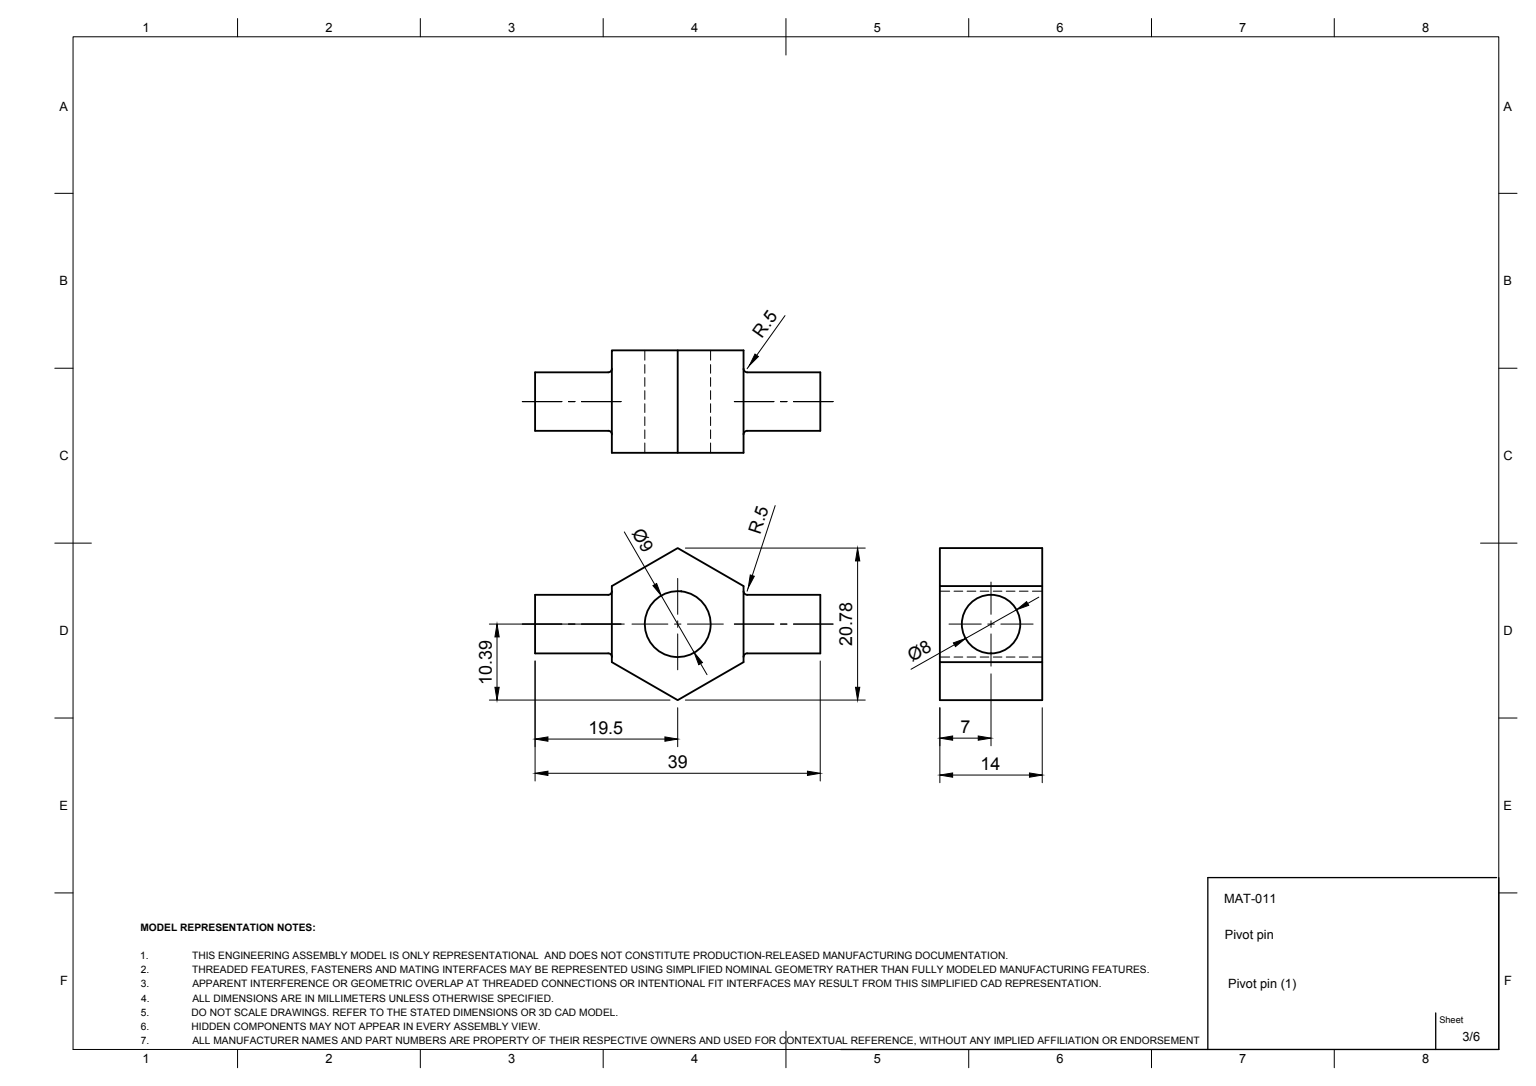
ISO-10303-21;
HEADER;
/* Generated by software containing ST-Developer
 * from STEP Tools, Inc. (www.steptools.com) 
 */

FILE_DESCRIPTION(
/* description */ ('STEP AP214'),
/* implementation_level */ '2;1');

FILE_NAME(
/* name */ 'Pivot Pin.step',
/* time_stamp */ '2026-11-14T05:56:09-08:00',
/* author */ (''),
/* organization */ (''),
/* preprocessor_version */ 'ST-DEVELOPER v20.2',
/* originating_system */ 'Autodesk Translation Framework v15.17.0.0',
/* authorisation */ '');

FILE_SCHEMA (('AUTOMOTIVE_DESIGN { 1 0 10303 214 3 1 1 }'));
ENDSEC;

DATA;
#10=MECHANICAL_DESIGN_GEOMETRIC_PRESENTATION_REPRESENTATION('',(#103),#3207);
#91=SHAPE_REPRESENTATION_RELATIONSHIP('SRR','None',#3243,#97);
#97=ADVANCED_BREP_SHAPE_REPRESENTATION('',(#109),#3202);
#103=STYLED_ITEM('',(#3282),#109);
#109=MANIFOLD_SOLID_BREP('Body1',#1281);
#121=PLANE('',#1388);
#122=PLANE('',#1389);
#123=PLANE('',#1390);
#124=PLANE('',#1391);
#125=PLANE('',#1392);
#126=PLANE('',#1393);
#127=PLANE('',#1394);
#128=PLANE('',#1395);
#129=PLANE('',#1396);
#130=PLANE('',#1397);
#163=LINE('',#2019,#230);
#164=LINE('',#2023,#231);
#165=LINE('',#2029,#232);
#166=LINE('',#2034,#233);
#167=LINE('',#2036,#234);
#168=LINE('',#2038,#235);
#169=LINE('',#2039,#236);
#170=LINE('',#2043,#237);
#171=LINE('',#2045,#238);
#172=LINE('',#2047,#239);
#173=LINE('',#2048,#240);
#174=LINE('',#2051,#241);
#175=LINE('',#2052,#242);
#176=LINE('',#2054,#243);
#177=LINE('',#2055,#244);
#178=LINE('',#2058,#245);
#179=LINE('',#2060,#246);
#180=LINE('',#2061,#247);
#181=LINE('',#2062,#248);
#182=LINE('',#2064,#249);
#183=LINE('',#2067,#250);
#230=VECTOR('',#1587,4.);
#231=VECTOR('',#1592,4.);
#232=VECTOR('',#1599,4.5);
#233=VECTOR('',#1604,1000.);
#234=VECTOR('',#1605,1000.);
#235=VECTOR('',#1606,1000.);
#236=VECTOR('',#1607,1000.);
#237=VECTOR('',#1610,1000.);
#238=VECTOR('',#1611,1000.);
#239=VECTOR('',#1612,1000.);
#240=VECTOR('',#1613,1000.);
#241=VECTOR('',#1616,1000.);
#242=VECTOR('',#1617,1000.);
#243=VECTOR('',#1618,1000.);
#244=VECTOR('',#1619,1000.);
#245=VECTOR('',#1622,1000.);
#246=VECTOR('',#1623,1000.);
#247=VECTOR('',#1624,1000.);
#248=VECTOR('',#1625,1000.);
#249=VECTOR('',#1628,1000.);
#250=VECTOR('',#1633,1000.);
#287=CYLINDRICAL_SURFACE('',#1381,4.);
#288=CYLINDRICAL_SURFACE('',#1383,4.);
#289=CYLINDRICAL_SURFACE('',#1385,4.5);
#310=FACE_BOUND('',#438,.T.);
#311=FACE_BOUND('',#440,.T.);
#312=FACE_BOUND('',#442,.T.);
#313=FACE_BOUND('',#444,.T.);
#355=FACE_OUTER_BOUND('',#432,.T.);
#356=FACE_OUTER_BOUND('',#433,.T.);
#357=FACE_OUTER_BOUND('',#434,.T.);
#358=FACE_OUTER_BOUND('',#435,.T.);
#359=FACE_OUTER_BOUND('',#436,.T.);
#360=FACE_OUTER_BOUND('',#437,.T.);
#361=FACE_OUTER_BOUND('',#439,.T.);
#362=FACE_OUTER_BOUND('',#441,.T.);
#363=FACE_OUTER_BOUND('',#443,.T.);
#364=FACE_OUTER_BOUND('',#445,.T.);
#365=FACE_OUTER_BOUND('',#446,.T.);
#366=FACE_OUTER_BOUND('',#447,.T.);
#367=FACE_OUTER_BOUND('',#448,.T.);
#368=FACE_OUTER_BOUND('',#449,.T.);
#369=FACE_OUTER_BOUND('',#450,.T.);
#432=EDGE_LOOP('',(#903,#904,#905,#906));
#433=EDGE_LOOP('',(#907,#908,#909,#910));
#434=EDGE_LOOP('',(#911,#912,#913,#914));
#435=EDGE_LOOP('',(#915,#916,#917,#918));
#436=EDGE_LOOP('',(#919,#920,#921,#922));
#437=EDGE_LOOP('',(#923,#924,#925,#926));
#438=EDGE_LOOP('',(#927));
#439=EDGE_LOOP('',(#928,#929,#930,#931));
#440=EDGE_LOOP('',(#932));
#441=EDGE_LOOP('',(#933,#934,#935,#936,#937,#938));
#442=EDGE_LOOP('',(#939));
#443=EDGE_LOOP('',(#940,#941,#942,#943,#944,#945));
#444=EDGE_LOOP('',(#946));
#445=EDGE_LOOP('',(#947,#948,#949,#950));
#446=EDGE_LOOP('',(#951,#952,#953,#954));
#447=EDGE_LOOP('',(#955,#956,#957,#958));
#448=EDGE_LOOP('',(#959,#960,#961,#962));
#449=EDGE_LOOP('',(#963));
#450=EDGE_LOOP('',(#964));
#525=CIRCLE('',#1374,4.5);
#526=CIRCLE('',#1375,0.5);
#527=CIRCLE('',#1376,4.);
#528=CIRCLE('',#1378,4.5);
#529=CIRCLE('',#1379,0.5);
#530=CIRCLE('',#1380,4.);
#531=CIRCLE('',#1382,4.);
#532=CIRCLE('',#1384,4.);
#533=CIRCLE('',#1386,4.5);
#534=CIRCLE('',#1387,4.5);
#599=VERTEX_POINT('',#2006);
#600=VERTEX_POINT('',#2008);
#601=VERTEX_POINT('',#2012);
#602=VERTEX_POINT('',#2014);
#603=VERTEX_POINT('',#2018);
#604=VERTEX_POINT('',#2022);
#605=VERTEX_POINT('',#2026);
#606=VERTEX_POINT('',#2028);
#607=VERTEX_POINT('',#2032);
#608=VERTEX_POINT('',#2033);
#609=VERTEX_POINT('',#2035);
#610=VERTEX_POINT('',#2037);
#611=VERTEX_POINT('',#2041);
#612=VERTEX_POINT('',#2042);
#613=VERTEX_POINT('',#2044);
#614=VERTEX_POINT('',#2046);
#615=VERTEX_POINT('',#2050);
#616=VERTEX_POINT('',#2053);
#617=VERTEX_POINT('',#2057);
#618=VERTEX_POINT('',#2059);
#715=EDGE_CURVE('',#599,#599,#525,.T.);
#716=EDGE_CURVE('',#599,#600,#526,.T.);
#717=EDGE_CURVE('',#600,#600,#527,.T.);
#718=EDGE_CURVE('',#601,#601,#528,.T.);
#719=EDGE_CURVE('',#601,#602,#529,.T.);
#720=EDGE_CURVE('',#602,#602,#530,.T.);
#721=EDGE_CURVE('',#600,#603,#163,.T.);
#722=EDGE_CURVE('',#603,#603,#531,.T.);
#723=EDGE_CURVE('',#602,#604,#164,.T.);
#724=EDGE_CURVE('',#604,#604,#532,.T.);
#725=EDGE_CURVE('',#605,#605,#533,.T.);
#726=EDGE_CURVE('',#605,#606,#165,.T.);
#727=EDGE_CURVE('',#606,#606,#534,.T.);
#728=EDGE_CURVE('',#607,#608,#166,.T.);
#729=EDGE_CURVE('',#609,#608,#167,.T.);
#730=EDGE_CURVE('',#610,#609,#168,.T.);
#731=EDGE_CURVE('',#610,#607,#169,.T.);
#732=EDGE_CURVE('',#611,#612,#170,.T.);
#733=EDGE_CURVE('',#613,#612,#171,.T.);
#734=EDGE_CURVE('',#614,#613,#172,.T.);
#735=EDGE_CURVE('',#614,#611,#173,.T.);
#736=EDGE_CURVE('',#609,#615,#174,.T.);
#737=EDGE_CURVE('',#615,#614,#175,.T.);
#738=EDGE_CURVE('',#613,#616,#176,.T.);
#739=EDGE_CURVE('',#616,#610,#177,.T.);
#740=EDGE_CURVE('',#608,#617,#178,.T.);
#741=EDGE_CURVE('',#618,#607,#179,.T.);
#742=EDGE_CURVE('',#612,#618,#180,.T.);
#743=EDGE_CURVE('',#617,#611,#181,.T.);
#744=EDGE_CURVE('',#615,#617,#182,.T.);
#745=EDGE_CURVE('',#616,#618,#183,.T.);
#903=ORIENTED_EDGE('',*,*,#715,.F.);
#904=ORIENTED_EDGE('',*,*,#716,.T.);
#905=ORIENTED_EDGE('',*,*,#717,.F.);
#906=ORIENTED_EDGE('',*,*,#716,.F.);
#907=ORIENTED_EDGE('',*,*,#718,.F.);
#908=ORIENTED_EDGE('',*,*,#719,.T.);
#909=ORIENTED_EDGE('',*,*,#720,.F.);
#910=ORIENTED_EDGE('',*,*,#719,.F.);
#911=ORIENTED_EDGE('',*,*,#717,.T.);
#912=ORIENTED_EDGE('',*,*,#721,.T.);
#913=ORIENTED_EDGE('',*,*,#722,.F.);
#914=ORIENTED_EDGE('',*,*,#721,.F.);
#915=ORIENTED_EDGE('',*,*,#720,.T.);
#916=ORIENTED_EDGE('',*,*,#723,.T.);
#917=ORIENTED_EDGE('',*,*,#724,.F.);
#918=ORIENTED_EDGE('',*,*,#723,.F.);
#919=ORIENTED_EDGE('',*,*,#725,.T.);
#920=ORIENTED_EDGE('',*,*,#726,.T.);
#921=ORIENTED_EDGE('',*,*,#727,.F.);
#922=ORIENTED_EDGE('',*,*,#726,.F.);
#923=ORIENTED_EDGE('',*,*,#728,.T.);
#924=ORIENTED_EDGE('',*,*,#729,.F.);
#925=ORIENTED_EDGE('',*,*,#730,.F.);
#926=ORIENTED_EDGE('',*,*,#731,.T.);
#927=ORIENTED_EDGE('',*,*,#715,.T.);
#928=ORIENTED_EDGE('',*,*,#732,.T.);
#929=ORIENTED_EDGE('',*,*,#733,.F.);
#930=ORIENTED_EDGE('',*,*,#734,.F.);
#931=ORIENTED_EDGE('',*,*,#735,.T.);
#932=ORIENTED_EDGE('',*,*,#718,.T.);
#933=ORIENTED_EDGE('',*,*,#736,.T.);
#934=ORIENTED_EDGE('',*,*,#737,.T.);
#935=ORIENTED_EDGE('',*,*,#734,.T.);
#936=ORIENTED_EDGE('',*,*,#738,.T.);
#937=ORIENTED_EDGE('',*,*,#739,.T.);
#938=ORIENTED_EDGE('',*,*,#730,.T.);
#939=ORIENTED_EDGE('',*,*,#725,.F.);
#940=ORIENTED_EDGE('',*,*,#740,.F.);
#941=ORIENTED_EDGE('',*,*,#728,.F.);
#942=ORIENTED_EDGE('',*,*,#741,.F.);
#943=ORIENTED_EDGE('',*,*,#742,.F.);
#944=ORIENTED_EDGE('',*,*,#732,.F.);
#945=ORIENTED_EDGE('',*,*,#743,.F.);
#946=ORIENTED_EDGE('',*,*,#727,.T.);
#947=ORIENTED_EDGE('',*,*,#740,.T.);
#948=ORIENTED_EDGE('',*,*,#744,.F.);
#949=ORIENTED_EDGE('',*,*,#736,.F.);
#950=ORIENTED_EDGE('',*,*,#729,.T.);
#951=ORIENTED_EDGE('',*,*,#743,.T.);
#952=ORIENTED_EDGE('',*,*,#735,.F.);
#953=ORIENTED_EDGE('',*,*,#737,.F.);
#954=ORIENTED_EDGE('',*,*,#744,.T.);
#955=ORIENTED_EDGE('',*,*,#742,.T.);
#956=ORIENTED_EDGE('',*,*,#745,.F.);
#957=ORIENTED_EDGE('',*,*,#738,.F.);
#958=ORIENTED_EDGE('',*,*,#733,.T.);
#959=ORIENTED_EDGE('',*,*,#741,.T.);
#960=ORIENTED_EDGE('',*,*,#731,.F.);
#961=ORIENTED_EDGE('',*,*,#739,.F.);
#962=ORIENTED_EDGE('',*,*,#745,.T.);
#963=ORIENTED_EDGE('',*,*,#724,.T.);
#964=ORIENTED_EDGE('',*,*,#722,.T.);
#1196=TOROIDAL_SURFACE('',#1373,4.5,0.5);
#1197=TOROIDAL_SURFACE('',#1377,4.5,0.5);
#1213=ADVANCED_FACE('',(#355),#1196,.F.);
#1214=ADVANCED_FACE('',(#356),#1197,.F.);
#1215=ADVANCED_FACE('',(#357),#287,.T.);
#1216=ADVANCED_FACE('',(#358),#288,.T.);
#1217=ADVANCED_FACE('',(#359),#289,.F.);
#1218=ADVANCED_FACE('',(#360,#310),#121,.F.);
#1219=ADVANCED_FACE('',(#361,#311),#122,.F.);
#1220=ADVANCED_FACE('',(#362,#312),#123,.T.);
#1221=ADVANCED_FACE('',(#363,#313),#124,.F.);
#1222=ADVANCED_FACE('',(#364),#125,.F.);
#1223=ADVANCED_FACE('',(#365),#126,.F.);
#1224=ADVANCED_FACE('',(#366),#127,.F.);
#1225=ADVANCED_FACE('',(#367),#128,.F.);
#1226=ADVANCED_FACE('',(#368),#129,.T.);
#1227=ADVANCED_FACE('',(#369),#130,.T.);
#1281=CLOSED_SHELL('',(#1213,#1214,#1215,#1216,#1217,#1218,#1219,#1220,
#1221,#1222,#1223,#1224,#1225,#1226,#1227));
#1372=AXIS2_PLACEMENT_3D('',#2004,#1567,#1568);
#1373=AXIS2_PLACEMENT_3D('',#2005,#1569,#1570);
#1374=AXIS2_PLACEMENT_3D('',#2007,#1571,#1572);
#1375=AXIS2_PLACEMENT_3D('',#2009,#1573,#1574);
#1376=AXIS2_PLACEMENT_3D('',#2010,#1575,#1576);
#1377=AXIS2_PLACEMENT_3D('',#2011,#1577,#1578);
#1378=AXIS2_PLACEMENT_3D('',#2013,#1579,#1580);
#1379=AXIS2_PLACEMENT_3D('',#2015,#1581,#1582);
#1380=AXIS2_PLACEMENT_3D('',#2016,#1583,#1584);
#1381=AXIS2_PLACEMENT_3D('',#2017,#1585,#1586);
#1382=AXIS2_PLACEMENT_3D('',#2020,#1588,#1589);
#1383=AXIS2_PLACEMENT_3D('',#2021,#1590,#1591);
#1384=AXIS2_PLACEMENT_3D('',#2024,#1593,#1594);
#1385=AXIS2_PLACEMENT_3D('',#2025,#1595,#1596);
#1386=AXIS2_PLACEMENT_3D('',#2027,#1597,#1598);
#1387=AXIS2_PLACEMENT_3D('',#2030,#1600,#1601);
#1388=AXIS2_PLACEMENT_3D('',#2031,#1602,#1603);
#1389=AXIS2_PLACEMENT_3D('',#2040,#1608,#1609);
#1390=AXIS2_PLACEMENT_3D('',#2049,#1614,#1615);
#1391=AXIS2_PLACEMENT_3D('',#2056,#1620,#1621);
#1392=AXIS2_PLACEMENT_3D('',#2063,#1626,#1627);
#1393=AXIS2_PLACEMENT_3D('',#2065,#1629,#1630);
#1394=AXIS2_PLACEMENT_3D('',#2066,#1631,#1632);
#1395=AXIS2_PLACEMENT_3D('',#2068,#1634,#1635);
#1396=AXIS2_PLACEMENT_3D('',#2069,#1636,#1637);
#1397=AXIS2_PLACEMENT_3D('',#2070,#1638,#1639);
#1567=DIRECTION('axis',(0.,0.,1.));
#1568=DIRECTION('refdir',(1.,0.,0.));
#1569=DIRECTION('center_axis',(3.33847688608258E-16,1.,0.));
#1570=DIRECTION('ref_axis',(-1.,3.5527136788005E-16,0.));
#1571=DIRECTION('center_axis',(3.33847688608258E-16,1.,0.));
#1572=DIRECTION('ref_axis',(-1.,3.33847688608258E-16,0.));
#1573=DIRECTION('center_axis',(2.22044604925031E-16,-7.41290781221554E-32,
1.));
#1574=DIRECTION('ref_axis',(1.,-4.44089209850063E-16,-2.22044604925031E-16));
#1575=DIRECTION('center_axis',(-3.33847688608258E-16,-1.,0.));
#1576=DIRECTION('ref_axis',(-1.,3.33847688608258E-16,0.));
#1577=DIRECTION('center_axis',(1.66923844304129E-16,-1.,0.));
#1578=DIRECTION('ref_axis',(1.,0.,0.));
#1579=DIRECTION('center_axis',(1.66923844304129E-16,-1.,0.));
#1580=DIRECTION('ref_axis',(1.,1.66923844304129E-16,0.));
#1581=DIRECTION('center_axis',(-2.22044604925031E-16,-3.70645390610778E-32,
1.));
#1582=DIRECTION('ref_axis',(-1.,-2.22044604925031E-16,-2.22044604925031E-16));
#1583=DIRECTION('center_axis',(-1.66923844304129E-16,1.,0.));
#1584=DIRECTION('ref_axis',(1.,1.66923844304129E-16,0.));
#1585=DIRECTION('center_axis',(3.33847688608258E-16,1.,0.));
#1586=DIRECTION('ref_axis',(-1.,3.33847688608258E-16,0.));
#1587=DIRECTION('',(-3.33847688608258E-16,-1.,0.));
#1588=DIRECTION('center_axis',(-3.33847688608258E-16,-1.,0.));
#1589=DIRECTION('ref_axis',(1.,-3.33847688608258E-16,0.));
#1590=DIRECTION('center_axis',(1.66923844304129E-16,-1.,0.));
#1591=DIRECTION('ref_axis',(1.,1.66923844304129E-16,0.));
#1592=DIRECTION('',(-1.66923844304129E-16,1.,0.));
#1593=DIRECTION('center_axis',(-1.66923844304129E-16,1.,0.));
#1594=DIRECTION('ref_axis',(-1.,-1.66923844304129E-16,0.));
#1595=DIRECTION('center_axis',(0.,0.,-1.));
#1596=DIRECTION('ref_axis',(-1.,0.,0.));
#1597=DIRECTION('center_axis',(0.,0.,1.));
#1598=DIRECTION('ref_axis',(1.,0.,0.));
#1599=DIRECTION('',(0.,0.,-1.));
#1600=DIRECTION('center_axis',(0.,0.,1.));
#1601=DIRECTION('ref_axis',(1.,0.,0.));
#1602=DIRECTION('center_axis',(3.33847688608258E-16,1.,0.));
#1603=DIRECTION('ref_axis',(-1.,3.33847688608258E-16,0.));
#1604=DIRECTION('',(1.,-3.33847688608257E-16,0.));
#1605=DIRECTION('',(0.,0.,-1.));
#1606=DIRECTION('',(1.,-3.33847688608257E-16,0.));
#1607=DIRECTION('',(0.,0.,-1.));
#1608=DIRECTION('center_axis',(1.66923844304129E-16,-1.,0.));
#1609=DIRECTION('ref_axis',(1.,1.66923844304129E-16,0.));
#1610=DIRECTION('',(-1.,-1.66923844304129E-16,0.));
#1611=DIRECTION('',(0.,0.,-1.));
#1612=DIRECTION('',(-1.,-1.66923844304129E-16,0.));
#1613=DIRECTION('',(0.,0.,-1.));
#1614=DIRECTION('center_axis',(0.,0.,1.));
#1615=DIRECTION('ref_axis',(1.,0.,0.));
#1616=DIRECTION('',(0.499999999999999,0.866025403784439,0.));
#1617=DIRECTION('',(-0.5,0.866025403784438,0.));
#1618=DIRECTION('',(-0.5,-0.866025403784439,0.));
#1619=DIRECTION('',(0.5,-0.866025403784439,0.));
#1620=DIRECTION('center_axis',(0.,0.,1.));
#1621=DIRECTION('ref_axis',(1.,0.,0.));
#1622=DIRECTION('',(0.499999999999999,0.866025403784439,0.));
#1623=DIRECTION('',(0.5,-0.866025403784439,0.));
#1624=DIRECTION('',(-0.5,-0.866025403784439,0.));
#1625=DIRECTION('',(-0.5,0.866025403784438,0.));
#1626=DIRECTION('center_axis',(-0.866025403784439,0.5,0.));
#1627=DIRECTION('ref_axis',(-0.5,-0.866025403784439,0.));
#1628=DIRECTION('',(0.,0.,-1.));
#1629=DIRECTION('center_axis',(-0.866025403784439,-0.5,0.));
#1630=DIRECTION('ref_axis',(0.5,-0.866025403784439,0.));
#1631=DIRECTION('center_axis',(0.866025403784439,-0.5,0.));
#1632=DIRECTION('ref_axis',(0.5,0.866025403784439,0.));
#1633=DIRECTION('',(0.,0.,-1.));
#1634=DIRECTION('center_axis',(0.866025403784439,0.5,0.));
#1635=DIRECTION('ref_axis',(-0.5,0.866025403784439,0.));
#1636=DIRECTION('center_axis',(-1.66923844304129E-16,1.,0.));
#1637=DIRECTION('ref_axis',(-1.,-1.66923844304129E-16,0.));
#1638=DIRECTION('center_axis',(-3.33847688608258E-16,-1.,0.));
#1639=DIRECTION('ref_axis',(1.,-3.33847688608258E-16,0.));
#2004=CARTESIAN_POINT('',(0.,0.,0.));
#2005=CARTESIAN_POINT('Origin',(-3.17155304177845E-15,-9.50000000000001,
7.));
#2006=CARTESIAN_POINT('',(4.5,-9.00000000000001,7.));
#2007=CARTESIAN_POINT('Origin',(-3.00462919747432E-15,-9.00000000000001,
7.));
#2008=CARTESIAN_POINT('',(4.,-9.50000000000001,7.));
#2009=CARTESIAN_POINT('Origin',(4.5,-9.50000000000001,7.));
#2010=CARTESIAN_POINT('Origin',(-3.17155304177845E-15,-9.50000000000001,
7.));
#2011=CARTESIAN_POINT('Origin',(-7.28523761486083E-16,9.50000000000003,
7.));
#2012=CARTESIAN_POINT('',(-4.5,9.00000000000002,7.));
#2013=CARTESIAN_POINT('Origin',(-6.45061839334019E-16,9.00000000000002,
7.));
#2014=CARTESIAN_POINT('',(-4.,9.50000000000002,7.));
#2015=CARTESIAN_POINT('Origin',(-4.5,9.50000000000003,7.));
#2016=CARTESIAN_POINT('Origin',(-7.28523761486083E-16,9.50000000000003,
7.));
#2017=CARTESIAN_POINT('Origin',(-6.51002992786103E-15,-19.5,7.));
#2018=CARTESIAN_POINT('',(3.99999999999999,-19.5,7.));
#2019=CARTESIAN_POINT('',(3.99999999999999,-19.5,7.));
#2020=CARTESIAN_POINT('Origin',(-6.51002992786103E-15,-19.5,7.));
#2021=CARTESIAN_POINT('Origin',(-2.39776220452737E-15,19.5,7.));
#2022=CARTESIAN_POINT('',(-4.,19.5,7.));
#2023=CARTESIAN_POINT('',(-4.,19.5,7.));
#2024=CARTESIAN_POINT('Origin',(-2.39776220452737E-15,19.5,7.));
#2025=CARTESIAN_POINT('Origin',(0.,0.,14.));
#2026=CARTESIAN_POINT('',(4.5,-5.51091059616309E-16,14.));
#2027=CARTESIAN_POINT('Origin',(0.,0.,14.));
#2028=CARTESIAN_POINT('',(4.5,-5.51091059616309E-16,0.));
#2029=CARTESIAN_POINT('',(4.5,-5.51091059616309E-16,14.));
#2030=CARTESIAN_POINT('Origin',(0.,0.,0.));
#2031=CARTESIAN_POINT('Origin',(-5.19615242270664,-9.00000000000001,14.));
#2032=CARTESIAN_POINT('',(-5.19615242270664,-9.00000000000001,0.));
#2033=CARTESIAN_POINT('',(5.19615242270663,-9.00000000000001,0.));
#2034=CARTESIAN_POINT('',(-5.19615242270664,-9.00000000000001,0.));
#2035=CARTESIAN_POINT('',(5.19615242270663,-9.00000000000001,14.));
#2036=CARTESIAN_POINT('',(5.19615242270663,-9.00000000000001,14.));
#2037=CARTESIAN_POINT('',(-5.19615242270664,-9.00000000000001,14.));
#2038=CARTESIAN_POINT('',(-5.19615242270664,-9.00000000000001,14.));
#2039=CARTESIAN_POINT('',(-5.19615242270664,-9.00000000000001,14.));
#2040=CARTESIAN_POINT('Origin',(5.19615242270661,9.00000000000002,14.));
#2041=CARTESIAN_POINT('',(5.19615242270661,9.00000000000002,0.));
#2042=CARTESIAN_POINT('',(-5.19615242270664,9.00000000000002,0.));
#2043=CARTESIAN_POINT('',(5.19615242270661,9.00000000000002,0.));
#2044=CARTESIAN_POINT('',(-5.19615242270664,9.00000000000002,14.));
#2045=CARTESIAN_POINT('',(-5.19615242270664,9.00000000000002,14.));
#2046=CARTESIAN_POINT('',(5.19615242270661,9.00000000000002,14.));
#2047=CARTESIAN_POINT('',(5.19615242270661,9.00000000000002,14.));
#2048=CARTESIAN_POINT('',(5.19615242270661,9.00000000000002,14.));
#2049=CARTESIAN_POINT('Origin',(0.,0.,14.));
#2050=CARTESIAN_POINT('',(10.3923048454133,7.03904010014224E-16,14.));
#2051=CARTESIAN_POINT('',(5.19615242270663,-9.00000000000001,14.));
#2052=CARTESIAN_POINT('',(10.3923048454133,7.03904010014224E-16,14.));
#2053=CARTESIAN_POINT('',(-10.3923048454133,-8.2724230250131E-16,14.));
#2054=CARTESIAN_POINT('',(-5.19615242270664,9.00000000000002,14.));
#2055=CARTESIAN_POINT('',(-10.3923048454133,-8.2724230250131E-16,14.));
#2056=CARTESIAN_POINT('Origin',(0.,0.,0.));
#2057=CARTESIAN_POINT('',(10.3923048454133,7.03904010014224E-16,0.));
#2058=CARTESIAN_POINT('',(5.19615242270663,-9.00000000000001,0.));
#2059=CARTESIAN_POINT('',(-10.3923048454133,-8.2724230250131E-16,0.));
#2060=CARTESIAN_POINT('',(-10.3923048454133,-8.2724230250131E-16,0.));
#2061=CARTESIAN_POINT('',(-5.19615242270664,9.00000000000002,0.));
#2062=CARTESIAN_POINT('',(10.3923048454133,7.03904010014224E-16,0.));
#2063=CARTESIAN_POINT('Origin',(5.19615242270663,-9.00000000000001,14.));
#2064=CARTESIAN_POINT('',(10.3923048454133,7.03904010014224E-16,14.));
#2065=CARTESIAN_POINT('Origin',(10.3923048454133,7.03904010014224E-16,14.));
#2066=CARTESIAN_POINT('Origin',(-5.19615242270664,9.00000000000002,14.));
#2067=CARTESIAN_POINT('',(-10.3923048454133,-8.2724230250131E-16,14.));
#2068=CARTESIAN_POINT('Origin',(-10.3923048454133,-8.2724230250131E-16,
14.));
#2069=CARTESIAN_POINT('Origin',(-2.39776220452737E-15,19.5,7.));
#2070=CARTESIAN_POINT('Origin',(-6.51002992786103E-15,-19.5,7.));
#3194=UNCERTAINTY_MEASURE_WITH_UNIT(LENGTH_MEASURE(0.01),#3208,
'DISTANCE_ACCURACY_VALUE',
'Maximum model space distance between geometric entities at asserted c
onnectivities');
#3199=UNCERTAINTY_MEASURE_WITH_UNIT(LENGTH_MEASURE(0.01),#3208,
'DISTANCE_ACCURACY_VALUE',
'Maximum model space distance between geometric entities at asserted c
onnectivities');
#3202=(
GEOMETRIC_REPRESENTATION_CONTEXT(3)
GLOBAL_UNCERTAINTY_ASSIGNED_CONTEXT((#3194))
GLOBAL_UNIT_ASSIGNED_CONTEXT((#3208,#3210,#3211))
REPRESENTATION_CONTEXT('','3D')
);
#3207=(
GEOMETRIC_REPRESENTATION_CONTEXT(3)
GLOBAL_UNCERTAINTY_ASSIGNED_CONTEXT((#3199))
GLOBAL_UNIT_ASSIGNED_CONTEXT((#3208,#3210,#3211))
REPRESENTATION_CONTEXT('','3D')
);
#3208=(
LENGTH_UNIT()
NAMED_UNIT(*)
SI_UNIT(.MILLI.,.METRE.)
);
#3210=(
NAMED_UNIT(*)
PLANE_ANGLE_UNIT()
SI_UNIT($,.RADIAN.)
);
#3211=(
NAMED_UNIT(*)
SI_UNIT($,.STERADIAN.)
SOLID_ANGLE_UNIT()
);
#3214=SHAPE_DEFINITION_REPRESENTATION(#3221,#3243);
#3221=PRODUCT_DEFINITION_SHAPE('',$,#3251);
#3243=SHAPE_REPRESENTATION('',(#1372),#3202);
#3248=PRODUCT_DEFINITION_CONTEXT('part definition',#3271,'design');
#3251=PRODUCT_DEFINITION('Pivot pin','Pivot Pin',#3258,#3248);
#3258=PRODUCT_DEFINITION_FORMATION('',$,#3275);
#3271=APPLICATION_CONTEXT(
'Core Data for Automotive Mechanical Design Process');
#3272=PRODUCT_CONTEXT('part definition',#3271,'mechanical');
#3275=PRODUCT('Pivot pin','Pivot Pin','Pivot pin',(#3272));
#3282=PRESENTATION_STYLE_ASSIGNMENT((#3286));
#3286=SURFACE_STYLE_USAGE(.BOTH.,#3290);
#3290=SURFACE_SIDE_STYLE('',(#3294));
#3294=SURFACE_STYLE_FILL_AREA(#3298);
#3298=FILL_AREA_STYLE('Opaque(227,224,212)',(#3302));
#3302=FILL_AREA_STYLE_COLOUR('Opaque(227,224,212)',#3306);
#3306=COLOUR_RGB('Opaque(227,224,212)',0.890196078431372,0.87843137254902,
0.831372549019608);
ENDSEC;
END-ISO-10303-21;
